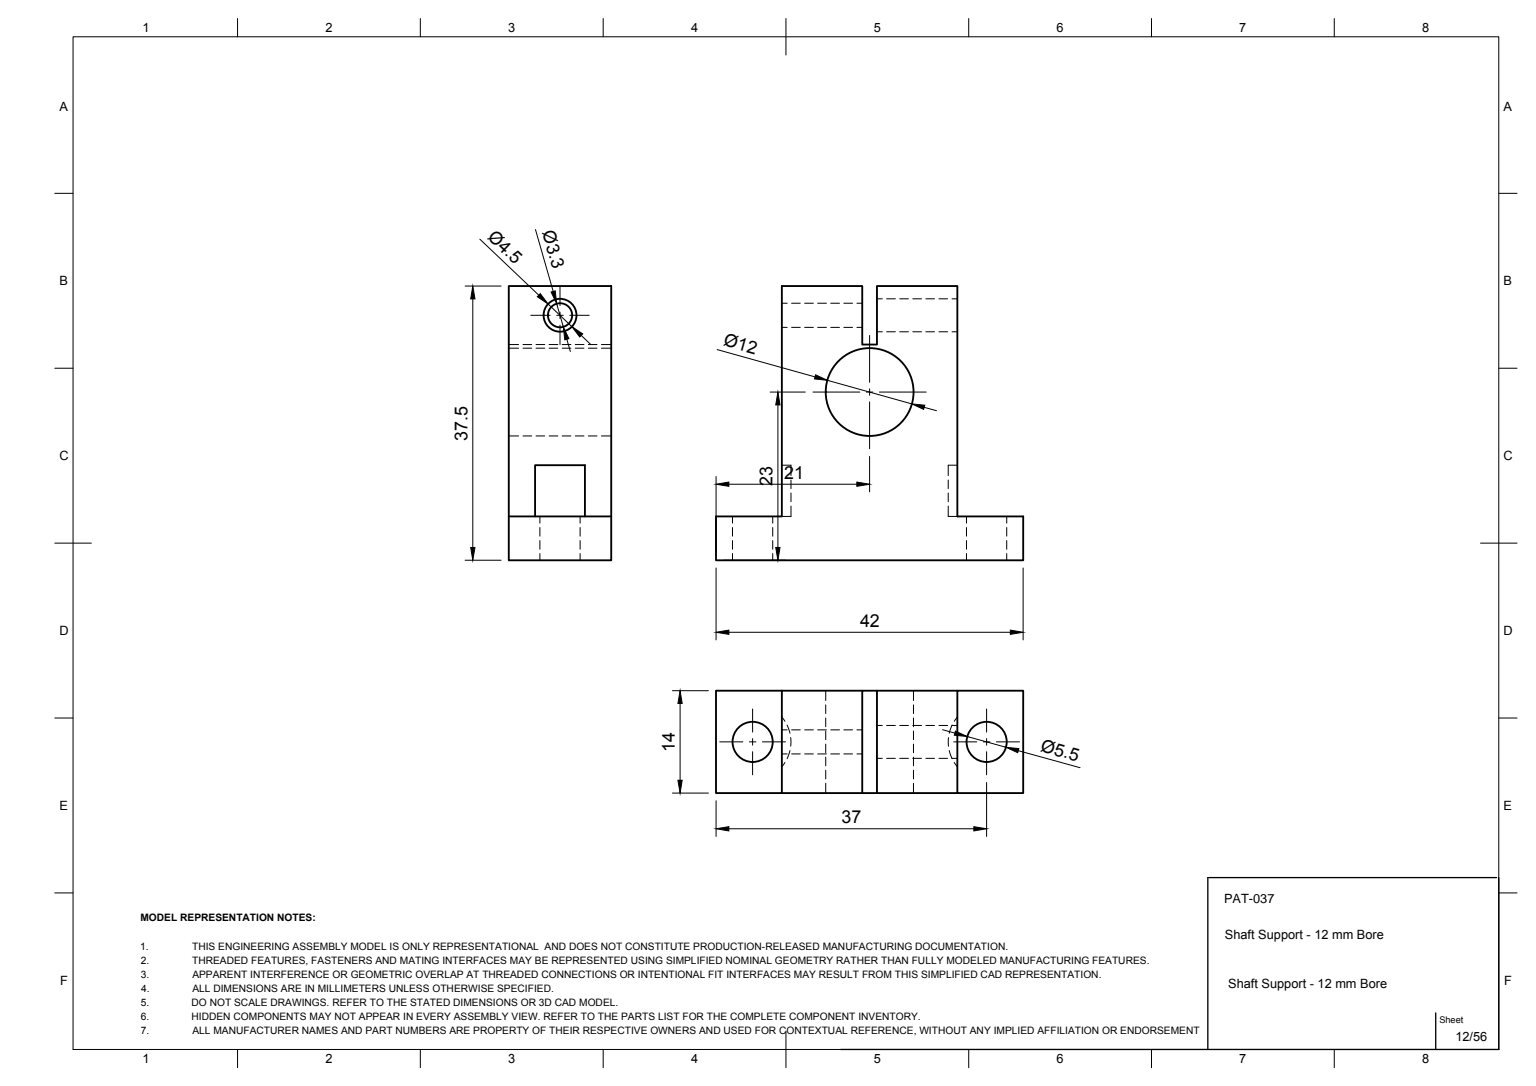
ISO-10303-21;
HEADER;
/* Generated by software containing ST-Developer
 * from STEP Tools, Inc. (www.steptools.com) 
 */

FILE_DESCRIPTION(
/* description */ ('Flywheel Crank-Slider'),
/* implementation_level */ '2;1');

FILE_NAME(
/* name */ 'Shaft Support - 12 mm Bore.step',
/* time_stamp */ '2026-10-28T03:23:13-07:00',
/* author */ (''),
/* organization */ (''),
/* preprocessor_version */ 'ST-DEVELOPER v20.2',
/* originating_system */ 'Autodesk Translation Framework v15.17.0.0',
/* authorisation */ '');

FILE_SCHEMA (('AUTOMOTIVE_DESIGN { 1 0 10303 214 3 1 1 }'));
ENDSEC;

DATA;
#10=MECHANICAL_DESIGN_GEOMETRIC_PRESENTATION_REPRESENTATION('',(#685),#17322);
#580=SHAPE_REPRESENTATION_RELATIONSHIP('SRR','None',#17577,#632);
#632=ADVANCED_BREP_SHAPE_REPRESENTATION('',(#744),#17281);
#685=STYLED_ITEM('',(#17931),#744);
#744=MANIFOLD_SOLID_BREP('Body1',#9065);
#894=FACE_BOUND('',#2179,.T.);
#895=FACE_BOUND('',#2181,.T.);
#896=FACE_BOUND('',#2183,.T.);
#897=FACE_BOUND('',#2190,.T.);
#898=FACE_BOUND('',#2193,.T.);
#899=FACE_BOUND('',#2194,.T.);
#900=FACE_BOUND('',#2197,.T.);
#901=FACE_BOUND('',#2200,.T.);
#902=FACE_BOUND('',#2203,.T.);
#903=FACE_BOUND('',#2206,.T.);
#1133=PLANE('',#10078);
#1134=PLANE('',#10085);
#1135=PLANE('',#10086);
#1136=PLANE('',#10088);
#1137=PLANE('',#10090);
#1138=PLANE('',#10104);
#1139=PLANE('',#10105);
#1140=PLANE('',#10106);
#1141=PLANE('',#10107);
#1142=PLANE('',#10108);
#1143=PLANE('',#10109);
#1144=PLANE('',#10110);
#1145=PLANE('',#10111);
#1146=PLANE('',#10112);
#1147=PLANE('',#10113);
#1148=PLANE('',#10114);
#1530=FACE_OUTER_BOUND('',#2174,.T.);
#1531=FACE_OUTER_BOUND('',#2175,.T.);
#1532=FACE_OUTER_BOUND('',#2176,.T.);
#1533=FACE_OUTER_BOUND('',#2177,.T.);
#1534=FACE_OUTER_BOUND('',#2178,.T.);
#1535=FACE_OUTER_BOUND('',#2180,.T.);
#1536=FACE_OUTER_BOUND('',#2182,.T.);
#1537=FACE_OUTER_BOUND('',#2184,.T.);
#1538=FACE_OUTER_BOUND('',#2185,.T.);
#1539=FACE_OUTER_BOUND('',#2186,.T.);
#1540=FACE_OUTER_BOUND('',#2187,.T.);
#1541=FACE_OUTER_BOUND('',#2188,.T.);
#1542=FACE_OUTER_BOUND('',#2189,.T.);
#1543=FACE_OUTER_BOUND('',#2191,.T.);
#1544=FACE_OUTER_BOUND('',#2192,.T.);
#1545=FACE_OUTER_BOUND('',#2195,.T.);
#1546=FACE_OUTER_BOUND('',#2196,.T.);
#1547=FACE_OUTER_BOUND('',#2198,.T.);
#1548=FACE_OUTER_BOUND('',#2199,.T.);
#1549=FACE_OUTER_BOUND('',#2201,.T.);
#1550=FACE_OUTER_BOUND('',#2202,.T.);
#1551=FACE_OUTER_BOUND('',#2204,.T.);
#1552=FACE_OUTER_BOUND('',#2205,.T.);
#2174=EDGE_LOOP('',(#7002,#7003));
#2175=EDGE_LOOP('',(#7004,#7005,#7006,#7007));
#2176=EDGE_LOOP('',(#7008,#7009,#7010,#7011));
#2177=EDGE_LOOP('',(#7012,#7013));
#2178=EDGE_LOOP('',(#7014,#7015,#7016,#7017,#7018,#7019));
#2179=EDGE_LOOP('',(#7020));
#2180=EDGE_LOOP('',(#7021,#7022,#7023,#7024,#7025,#7026,#7027,#7028));
#2181=EDGE_LOOP('',(#7029));
#2182=EDGE_LOOP('',(#7030,#7031,#7032,#7033,#7034,#7035));
#2183=EDGE_LOOP('',(#7036));
#2184=EDGE_LOOP('',(#7037,#7038,#7039,#7040));
#2185=EDGE_LOOP('',(#7041,#7042,#7043,#7044));
#2186=EDGE_LOOP('',(#7045,#7046,#7047,#7048));
#2187=EDGE_LOOP('',(#7049,#7050,#7051,#7052));
#2188=EDGE_LOOP('',(#7053,#7054,#7055,#7056));
#2189=EDGE_LOOP('',(#7057,#7058,#7059,#7060,#7061,#7062,#7063,#7064,#7065,
#7066,#7067,#7068));
#2190=EDGE_LOOP('',(#7069));
#2191=EDGE_LOOP('',(#7070,#7071,#7072,#7073));
#2192=EDGE_LOOP('',(#7074,#7075,#7076,#7077));
#2193=EDGE_LOOP('',(#7078));
#2194=EDGE_LOOP('',(#7079));
#2195=EDGE_LOOP('',(#7080,#7081,#7082,#7083));
#2196=EDGE_LOOP('',(#7084,#7085,#7086,#7087,#7088,#7089,#7090,#7091));
#2197=EDGE_LOOP('',(#7092));
#2198=EDGE_LOOP('',(#7093,#7094,#7095,#7096));
#2199=EDGE_LOOP('',(#7097,#7098,#7099,#7100));
#2200=EDGE_LOOP('',(#7101));
#2201=EDGE_LOOP('',(#7102,#7103,#7104,#7105));
#2202=EDGE_LOOP('',(#7106,#7107,#7108,#7109));
#2203=EDGE_LOOP('',(#7110));
#2204=EDGE_LOOP('',(#7111,#7112,#7113,#7114));
#2205=EDGE_LOOP('',(#7115,#7116,#7117,#7118,#7119,#7120,#7121,#7122,#7123,
#7124,#7125,#7126));
#2206=EDGE_LOOP('',(#7127));
#2871=LINE('',#15107,#3482);
#2872=LINE('',#15111,#3483);
#2873=LINE('',#15114,#3484);
#2874=LINE('',#15118,#3485);
#2875=LINE('',#15122,#3486);
#2876=LINE('',#15125,#3487);
#2877=LINE('',#15128,#3488);
#2878=LINE('',#15130,#3489);
#2879=LINE('',#15132,#3490);
#2880=LINE('',#15134,#3491);
#2881=LINE('',#15135,#3492);
#2882=LINE('',#15140,#3493);
#2883=LINE('',#15142,#3494);
#2884=LINE('',#15143,#3495);
#2885=LINE('',#15149,#3496);
#2886=LINE('',#15151,#3497);
#2887=LINE('',#15152,#3498);
#2888=LINE('',#15154,#3499);
#2889=LINE('',#15155,#3500);
#2890=LINE('',#15162,#3501);
#2891=LINE('',#15166,#3502);
#2892=LINE('',#15171,#3503);
#2893=LINE('',#15175,#3504);
#2894=LINE('',#15180,#3505);
#2895=LINE('',#15184,#3506);
#2896=LINE('',#15186,#3507);
#2897=LINE('',#15187,#3508);
#2898=LINE('',#15189,#3509);
#2899=LINE('',#15191,#3510);
#2900=LINE('',#15193,#3511);
#2901=LINE('',#15195,#3512);
#2902=LINE('',#15197,#3513);
#2903=LINE('',#15198,#3514);
#2904=LINE('',#15201,#3515);
#2905=LINE('',#15202,#3516);
#2906=LINE('',#15205,#3517);
#2907=LINE('',#15206,#3518);
#2908=LINE('',#15208,#3519);
#2909=LINE('',#15211,#3520);
#2910=LINE('',#15212,#3521);
#2911=LINE('',#15215,#3522);
#2912=LINE('',#15216,#3523);
#2913=LINE('',#15219,#3524);
#2914=LINE('',#15220,#3525);
#2915=LINE('',#15223,#3526);
#2916=LINE('',#15224,#3527);
#2917=LINE('',#15227,#3528);
#2918=LINE('',#15228,#3529);
#2919=LINE('',#15230,#3530);
#3482=VECTOR('',#11873,1.);
#3483=VECTOR('',#11878,1.);
#3484=VECTOR('',#11881,1.);
#3485=VECTOR('',#11884,1.);
#3486=VECTOR('',#11887,1.);
#3487=VECTOR('',#11892,1.);
#3488=VECTOR('',#11895,1.);
#3489=VECTOR('',#11896,1.);
#3490=VECTOR('',#11897,1.);
#3491=VECTOR('',#11898,1.);
#3492=VECTOR('',#11899,1.);
#3493=VECTOR('',#11904,1.);
#3494=VECTOR('',#11905,1.);
#3495=VECTOR('',#11906,1.);
#3496=VECTOR('',#11911,1.);
#3497=VECTOR('',#11912,1.);
#3498=VECTOR('',#11913,1.);
#3499=VECTOR('',#11914,1.);
#3500=VECTOR('',#11915,1.);
#3501=VECTOR('',#11922,0.225);
#3502=VECTOR('',#11927,0.165);
#3503=VECTOR('',#11934,0.275);
#3504=VECTOR('',#11939,0.275);
#3505=VECTOR('',#11944,0.6);
#3506=VECTOR('',#11949,1.);
#3507=VECTOR('',#11950,1.);
#3508=VECTOR('',#11951,1.);
#3509=VECTOR('',#11952,1.);
#3510=VECTOR('',#11953,1.);
#3511=VECTOR('',#11954,1.);
#3512=VECTOR('',#11955,1.);
#3513=VECTOR('',#11956,1.);
#3514=VECTOR('',#11957,1.);
#3515=VECTOR('',#11960,1.);
#3516=VECTOR('',#11961,1.);
#3517=VECTOR('',#11964,1.);
#3518=VECTOR('',#11965,1.);
#3519=VECTOR('',#11968,1.);
#3520=VECTOR('',#11971,1.);
#3521=VECTOR('',#11972,1.);
#3522=VECTOR('',#11975,1.);
#3523=VECTOR('',#11976,1.);
#3524=VECTOR('',#11979,1.);
#3525=VECTOR('',#11980,1.);
#3526=VECTOR('',#11983,1.);
#3527=VECTOR('',#11984,1.);
#3528=VECTOR('',#11987,1.);
#3529=VECTOR('',#11988,1.);
#3530=VECTOR('',#11991,1.);
#3999=CIRCLE('',#10079,0.525);
#4000=CIRCLE('',#10081,0.525);
#4001=CIRCLE('',#10083,0.525);
#4002=CIRCLE('',#10084,0.525);
#4003=CIRCLE('',#10087,0.275);
#4004=CIRCLE('',#10089,0.165);
#4005=CIRCLE('',#10091,0.275);
#4006=CIRCLE('',#10093,0.225);
#4007=CIRCLE('',#10094,0.225);
#4008=CIRCLE('',#10096,0.165);
#4009=CIRCLE('',#10098,0.275);
#4010=CIRCLE('',#10100,0.275);
#4011=CIRCLE('',#10102,0.6);
#4012=CIRCLE('',#10103,0.6);
#4570=VERTEX_POINT('',#15105);
#4571=VERTEX_POINT('',#15106);
#4572=VERTEX_POINT('',#15110);
#4573=VERTEX_POINT('',#15112);
#4574=VERTEX_POINT('',#15116);
#4575=VERTEX_POINT('',#15117);
#4576=VERTEX_POINT('',#15119);
#4577=VERTEX_POINT('',#15121);
#4578=VERTEX_POINT('',#15127);
#4579=VERTEX_POINT('',#15129);
#4580=VERTEX_POINT('',#15131);
#4581=VERTEX_POINT('',#15133);
#4582=VERTEX_POINT('',#15136);
#4583=VERTEX_POINT('',#15139);
#4584=VERTEX_POINT('',#15141);
#4585=VERTEX_POINT('',#15144);
#4586=VERTEX_POINT('',#15147);
#4587=VERTEX_POINT('',#15148);
#4588=VERTEX_POINT('',#15150);
#4589=VERTEX_POINT('',#15153);
#4590=VERTEX_POINT('',#15156);
#4591=VERTEX_POINT('',#15159);
#4592=VERTEX_POINT('',#15161);
#4593=VERTEX_POINT('',#15165);
#4594=VERTEX_POINT('',#15169);
#4595=VERTEX_POINT('',#15173);
#4596=VERTEX_POINT('',#15177);
#4597=VERTEX_POINT('',#15179);
#4598=VERTEX_POINT('',#15183);
#4599=VERTEX_POINT('',#15185);
#4600=VERTEX_POINT('',#15188);
#4601=VERTEX_POINT('',#15190);
#4602=VERTEX_POINT('',#15192);
#4603=VERTEX_POINT('',#15194);
#4604=VERTEX_POINT('',#15196);
#4605=VERTEX_POINT('',#15200);
#4606=VERTEX_POINT('',#15204);
#4607=VERTEX_POINT('',#15210);
#4608=VERTEX_POINT('',#15214);
#4609=VERTEX_POINT('',#15218);
#4610=VERTEX_POINT('',#15222);
#4611=VERTEX_POINT('',#15226);
#5458=EDGE_CURVE('',#4570,#4571,#2871,.T.);
#5459=EDGE_CURVE('',#4571,#4570,#3999,.T.);
#5460=EDGE_CURVE('',#4572,#4570,#2872,.T.);
#5461=EDGE_CURVE('',#4573,#4572,#4000,.T.);
#5462=EDGE_CURVE('',#4571,#4573,#2873,.T.);
#5463=EDGE_CURVE('',#4574,#4575,#2874,.T.);
#5464=EDGE_CURVE('',#4574,#4576,#4001,.T.);
#5465=EDGE_CURVE('',#4577,#4576,#2875,.T.);
#5466=EDGE_CURVE('',#4575,#4577,#4002,.T.);
#5467=EDGE_CURVE('',#4576,#4574,#2876,.T.);
#5468=EDGE_CURVE('',#4572,#4578,#2877,.T.);
#5469=EDGE_CURVE('',#4579,#4578,#2878,.T.);
#5470=EDGE_CURVE('',#4579,#4580,#2879,.T.);
#5471=EDGE_CURVE('',#4581,#4580,#2880,.T.);
#5472=EDGE_CURVE('',#4581,#4573,#2881,.T.);
#5473=EDGE_CURVE('',#4582,#4582,#4003,.T.);
#5474=EDGE_CURVE('',#4583,#4581,#2882,.T.);
#5475=EDGE_CURVE('',#4583,#4584,#2883,.T.);
#5476=EDGE_CURVE('',#4578,#4584,#2884,.T.);
#5477=EDGE_CURVE('',#4585,#4585,#4004,.T.);
#5478=EDGE_CURVE('',#4586,#4587,#2885,.T.);
#5479=EDGE_CURVE('',#4588,#4587,#2886,.T.);
#5480=EDGE_CURVE('',#4575,#4588,#2887,.T.);
#5481=EDGE_CURVE('',#4589,#4577,#2888,.T.);
#5482=EDGE_CURVE('',#4586,#4589,#2889,.T.);
#5483=EDGE_CURVE('',#4590,#4590,#4005,.T.);
#5484=EDGE_CURVE('',#4591,#4591,#4006,.T.);
#5485=EDGE_CURVE('',#4591,#4592,#2890,.T.);
#5486=EDGE_CURVE('',#4592,#4592,#4007,.T.);
#5487=EDGE_CURVE('',#4585,#4593,#2891,.T.);
#5488=EDGE_CURVE('',#4593,#4593,#4008,.T.);
#5489=EDGE_CURVE('',#4594,#4594,#4009,.T.);
#5490=EDGE_CURVE('',#4594,#4582,#2892,.T.);
#5491=EDGE_CURVE('',#4595,#4595,#4010,.T.);
#5492=EDGE_CURVE('',#4595,#4590,#2893,.T.);
#5493=EDGE_CURVE('',#4596,#4596,#4011,.T.);
#5494=EDGE_CURVE('',#4596,#4597,#2894,.T.);
#5495=EDGE_CURVE('',#4597,#4597,#4012,.T.);
#5496=EDGE_CURVE('',#4580,#4598,#2895,.T.);
#5497=EDGE_CURVE('',#4598,#4599,#2896,.T.);
#5498=EDGE_CURVE('',#4599,#4586,#2897,.T.);
#5499=EDGE_CURVE('',#4589,#4600,#2898,.T.);
#5500=EDGE_CURVE('',#4600,#4601,#2899,.T.);
#5501=EDGE_CURVE('',#4601,#4602,#2900,.T.);
#5502=EDGE_CURVE('',#4602,#4603,#2901,.T.);
#5503=EDGE_CURVE('',#4603,#4604,#2902,.T.);
#5504=EDGE_CURVE('',#4604,#4583,#2903,.T.);
#5505=EDGE_CURVE('',#4605,#4579,#2904,.T.);
#5506=EDGE_CURVE('',#4598,#4605,#2905,.T.);
#5507=EDGE_CURVE('',#4606,#4605,#2906,.T.);
#5508=EDGE_CURVE('',#4599,#4606,#2907,.T.);
#5509=EDGE_CURVE('',#4587,#4606,#2908,.T.);
#5510=EDGE_CURVE('',#4607,#4588,#2909,.T.);
#5511=EDGE_CURVE('',#4600,#4607,#2910,.T.);
#5512=EDGE_CURVE('',#4608,#4607,#2911,.T.);
#5513=EDGE_CURVE('',#4601,#4608,#2912,.T.);
#5514=EDGE_CURVE('',#4609,#4608,#2913,.T.);
#5515=EDGE_CURVE('',#4602,#4609,#2914,.T.);
#5516=EDGE_CURVE('',#4610,#4609,#2915,.T.);
#5517=EDGE_CURVE('',#4603,#4610,#2916,.T.);
#5518=EDGE_CURVE('',#4611,#4610,#2917,.T.);
#5519=EDGE_CURVE('',#4604,#4611,#2918,.T.);
#5520=EDGE_CURVE('',#4584,#4611,#2919,.T.);
#7002=ORIENTED_EDGE('',*,*,#5458,.F.);
#7003=ORIENTED_EDGE('',*,*,#5459,.F.);
#7004=ORIENTED_EDGE('',*,*,#5460,.F.);
#7005=ORIENTED_EDGE('',*,*,#5461,.F.);
#7006=ORIENTED_EDGE('',*,*,#5462,.F.);
#7007=ORIENTED_EDGE('',*,*,#5459,.T.);
#7008=ORIENTED_EDGE('',*,*,#5463,.F.);
#7009=ORIENTED_EDGE('',*,*,#5464,.T.);
#7010=ORIENTED_EDGE('',*,*,#5465,.F.);
#7011=ORIENTED_EDGE('',*,*,#5466,.F.);
#7012=ORIENTED_EDGE('',*,*,#5467,.F.);
#7013=ORIENTED_EDGE('',*,*,#5464,.F.);
#7014=ORIENTED_EDGE('',*,*,#5468,.T.);
#7015=ORIENTED_EDGE('',*,*,#5469,.F.);
#7016=ORIENTED_EDGE('',*,*,#5470,.T.);
#7017=ORIENTED_EDGE('',*,*,#5471,.F.);
#7018=ORIENTED_EDGE('',*,*,#5472,.T.);
#7019=ORIENTED_EDGE('',*,*,#5461,.T.);
#7020=ORIENTED_EDGE('',*,*,#5473,.T.);
#7021=ORIENTED_EDGE('',*,*,#5460,.T.);
#7022=ORIENTED_EDGE('',*,*,#5458,.T.);
#7023=ORIENTED_EDGE('',*,*,#5462,.T.);
#7024=ORIENTED_EDGE('',*,*,#5472,.F.);
#7025=ORIENTED_EDGE('',*,*,#5474,.F.);
#7026=ORIENTED_EDGE('',*,*,#5475,.T.);
#7027=ORIENTED_EDGE('',*,*,#5476,.F.);
#7028=ORIENTED_EDGE('',*,*,#5468,.F.);
#7029=ORIENTED_EDGE('',*,*,#5477,.T.);
#7030=ORIENTED_EDGE('',*,*,#5478,.T.);
#7031=ORIENTED_EDGE('',*,*,#5479,.F.);
#7032=ORIENTED_EDGE('',*,*,#5480,.F.);
#7033=ORIENTED_EDGE('',*,*,#5466,.T.);
#7034=ORIENTED_EDGE('',*,*,#5481,.F.);
#7035=ORIENTED_EDGE('',*,*,#5482,.F.);
#7036=ORIENTED_EDGE('',*,*,#5483,.T.);
#7037=ORIENTED_EDGE('',*,*,#5484,.F.);
#7038=ORIENTED_EDGE('',*,*,#5485,.T.);
#7039=ORIENTED_EDGE('',*,*,#5486,.F.);
#7040=ORIENTED_EDGE('',*,*,#5485,.F.);
#7041=ORIENTED_EDGE('',*,*,#5477,.F.);
#7042=ORIENTED_EDGE('',*,*,#5487,.T.);
#7043=ORIENTED_EDGE('',*,*,#5488,.F.);
#7044=ORIENTED_EDGE('',*,*,#5487,.F.);
#7045=ORIENTED_EDGE('',*,*,#5489,.F.);
#7046=ORIENTED_EDGE('',*,*,#5490,.T.);
#7047=ORIENTED_EDGE('',*,*,#5473,.F.);
#7048=ORIENTED_EDGE('',*,*,#5490,.F.);
#7049=ORIENTED_EDGE('',*,*,#5491,.F.);
#7050=ORIENTED_EDGE('',*,*,#5492,.T.);
#7051=ORIENTED_EDGE('',*,*,#5483,.F.);
#7052=ORIENTED_EDGE('',*,*,#5492,.F.);
#7053=ORIENTED_EDGE('',*,*,#5493,.F.);
#7054=ORIENTED_EDGE('',*,*,#5494,.T.);
#7055=ORIENTED_EDGE('',*,*,#5495,.F.);
#7056=ORIENTED_EDGE('',*,*,#5494,.F.);
#7057=ORIENTED_EDGE('',*,*,#5471,.T.);
#7058=ORIENTED_EDGE('',*,*,#5496,.T.);
#7059=ORIENTED_EDGE('',*,*,#5497,.T.);
#7060=ORIENTED_EDGE('',*,*,#5498,.T.);
#7061=ORIENTED_EDGE('',*,*,#5482,.T.);
#7062=ORIENTED_EDGE('',*,*,#5499,.T.);
#7063=ORIENTED_EDGE('',*,*,#5500,.T.);
#7064=ORIENTED_EDGE('',*,*,#5501,.T.);
#7065=ORIENTED_EDGE('',*,*,#5502,.T.);
#7066=ORIENTED_EDGE('',*,*,#5503,.T.);
#7067=ORIENTED_EDGE('',*,*,#5504,.T.);
#7068=ORIENTED_EDGE('',*,*,#5474,.T.);
#7069=ORIENTED_EDGE('',*,*,#5493,.T.);
#7070=ORIENTED_EDGE('',*,*,#5470,.F.);
#7071=ORIENTED_EDGE('',*,*,#5505,.F.);
#7072=ORIENTED_EDGE('',*,*,#5506,.F.);
#7073=ORIENTED_EDGE('',*,*,#5496,.F.);
#7074=ORIENTED_EDGE('',*,*,#5506,.T.);
#7075=ORIENTED_EDGE('',*,*,#5507,.F.);
#7076=ORIENTED_EDGE('',*,*,#5508,.F.);
#7077=ORIENTED_EDGE('',*,*,#5497,.F.);
#7078=ORIENTED_EDGE('',*,*,#5489,.T.);
#7079=ORIENTED_EDGE('',*,*,#5491,.T.);
#7080=ORIENTED_EDGE('',*,*,#5508,.T.);
#7081=ORIENTED_EDGE('',*,*,#5509,.F.);
#7082=ORIENTED_EDGE('',*,*,#5478,.F.);
#7083=ORIENTED_EDGE('',*,*,#5498,.F.);
#7084=ORIENTED_EDGE('',*,*,#5463,.T.);
#7085=ORIENTED_EDGE('',*,*,#5480,.T.);
#7086=ORIENTED_EDGE('',*,*,#5510,.F.);
#7087=ORIENTED_EDGE('',*,*,#5511,.F.);
#7088=ORIENTED_EDGE('',*,*,#5499,.F.);
#7089=ORIENTED_EDGE('',*,*,#5481,.T.);
#7090=ORIENTED_EDGE('',*,*,#5465,.T.);
#7091=ORIENTED_EDGE('',*,*,#5467,.T.);
#7092=ORIENTED_EDGE('',*,*,#5486,.T.);
#7093=ORIENTED_EDGE('',*,*,#5511,.T.);
#7094=ORIENTED_EDGE('',*,*,#5512,.F.);
#7095=ORIENTED_EDGE('',*,*,#5513,.F.);
#7096=ORIENTED_EDGE('',*,*,#5500,.F.);
#7097=ORIENTED_EDGE('',*,*,#5513,.T.);
#7098=ORIENTED_EDGE('',*,*,#5514,.F.);
#7099=ORIENTED_EDGE('',*,*,#5515,.F.);
#7100=ORIENTED_EDGE('',*,*,#5501,.F.);
#7101=ORIENTED_EDGE('',*,*,#5484,.T.);
#7102=ORIENTED_EDGE('',*,*,#5515,.T.);
#7103=ORIENTED_EDGE('',*,*,#5516,.F.);
#7104=ORIENTED_EDGE('',*,*,#5517,.F.);
#7105=ORIENTED_EDGE('',*,*,#5502,.F.);
#7106=ORIENTED_EDGE('',*,*,#5517,.T.);
#7107=ORIENTED_EDGE('',*,*,#5518,.F.);
#7108=ORIENTED_EDGE('',*,*,#5519,.F.);
#7109=ORIENTED_EDGE('',*,*,#5503,.F.);
#7110=ORIENTED_EDGE('',*,*,#5488,.T.);
#7111=ORIENTED_EDGE('',*,*,#5519,.T.);
#7112=ORIENTED_EDGE('',*,*,#5520,.F.);
#7113=ORIENTED_EDGE('',*,*,#5475,.F.);
#7114=ORIENTED_EDGE('',*,*,#5504,.F.);
#7115=ORIENTED_EDGE('',*,*,#5469,.T.);
#7116=ORIENTED_EDGE('',*,*,#5476,.T.);
#7117=ORIENTED_EDGE('',*,*,#5520,.T.);
#7118=ORIENTED_EDGE('',*,*,#5518,.T.);
#7119=ORIENTED_EDGE('',*,*,#5516,.T.);
#7120=ORIENTED_EDGE('',*,*,#5514,.T.);
#7121=ORIENTED_EDGE('',*,*,#5512,.T.);
#7122=ORIENTED_EDGE('',*,*,#5510,.T.);
#7123=ORIENTED_EDGE('',*,*,#5479,.T.);
#7124=ORIENTED_EDGE('',*,*,#5509,.T.);
#7125=ORIENTED_EDGE('',*,*,#5507,.T.);
#7126=ORIENTED_EDGE('',*,*,#5505,.T.);
#7127=ORIENTED_EDGE('',*,*,#5495,.T.);
#8409=CYLINDRICAL_SURFACE('',#10080,0.525);
#8410=CYLINDRICAL_SURFACE('',#10082,0.525);
#8411=CYLINDRICAL_SURFACE('',#10092,0.225);
#8412=CYLINDRICAL_SURFACE('',#10095,0.165);
#8413=CYLINDRICAL_SURFACE('',#10097,0.275);
#8414=CYLINDRICAL_SURFACE('',#10099,0.275);
#8415=CYLINDRICAL_SURFACE('',#10101,0.6);
#8721=ADVANCED_FACE('',(#1530),#1133,.F.);
#8722=ADVANCED_FACE('',(#1531),#8409,.F.);
#8723=ADVANCED_FACE('',(#1532),#8410,.F.);
#8724=ADVANCED_FACE('',(#1533),#1134,.F.);
#8725=ADVANCED_FACE('',(#1534,#894),#1135,.T.);
#8726=ADVANCED_FACE('',(#1535,#895),#1136,.T.);
#8727=ADVANCED_FACE('',(#1536,#896),#1137,.T.);
#8728=ADVANCED_FACE('',(#1537),#8411,.F.);
#8729=ADVANCED_FACE('',(#1538),#8412,.F.);
#8730=ADVANCED_FACE('',(#1539),#8413,.F.);
#8731=ADVANCED_FACE('',(#1540),#8414,.F.);
#8732=ADVANCED_FACE('',(#1541),#8415,.F.);
#8733=ADVANCED_FACE('',(#1542,#897),#1138,.T.);
#8734=ADVANCED_FACE('',(#1543),#1139,.T.);
#8735=ADVANCED_FACE('',(#1544,#898,#899),#1140,.T.);
#8736=ADVANCED_FACE('',(#1545),#1141,.T.);
#8737=ADVANCED_FACE('',(#1546,#900),#1142,.T.);
#8738=ADVANCED_FACE('',(#1547),#1143,.T.);
#8739=ADVANCED_FACE('',(#1548,#901),#1144,.T.);
#8740=ADVANCED_FACE('',(#1549),#1145,.T.);
#8741=ADVANCED_FACE('',(#1550,#902),#1146,.T.);
#8742=ADVANCED_FACE('',(#1551),#1147,.T.);
#8743=ADVANCED_FACE('',(#1552,#903),#1148,.T.);
#9065=CLOSED_SHELL('',(#8721,#8722,#8723,#8724,#8725,#8726,#8727,#8728,
#8729,#8730,#8731,#8732,#8733,#8734,#8735,#8736,#8737,#8738,#8739,#8740,
#8741,#8742,#8743));
#10077=AXIS2_PLACEMENT_3D('',#15103,#11869,#11870);
#10078=AXIS2_PLACEMENT_3D('',#15104,#11871,#11872);
#10079=AXIS2_PLACEMENT_3D('',#15108,#11874,#11875);
#10080=AXIS2_PLACEMENT_3D('',#15109,#11876,#11877);
#10081=AXIS2_PLACEMENT_3D('',#15113,#11879,#11880);
#10082=AXIS2_PLACEMENT_3D('',#15115,#11882,#11883);
#10083=AXIS2_PLACEMENT_3D('',#15120,#11885,#11886);
#10084=AXIS2_PLACEMENT_3D('',#15123,#11888,#11889);
#10085=AXIS2_PLACEMENT_3D('',#15124,#11890,#11891);
#10086=AXIS2_PLACEMENT_3D('',#15126,#11893,#11894);
#10087=AXIS2_PLACEMENT_3D('',#15137,#11900,#11901);
#10088=AXIS2_PLACEMENT_3D('',#15138,#11902,#11903);
#10089=AXIS2_PLACEMENT_3D('',#15145,#11907,#11908);
#10090=AXIS2_PLACEMENT_3D('',#15146,#11909,#11910);
#10091=AXIS2_PLACEMENT_3D('',#15157,#11916,#11917);
#10092=AXIS2_PLACEMENT_3D('',#15158,#11918,#11919);
#10093=AXIS2_PLACEMENT_3D('',#15160,#11920,#11921);
#10094=AXIS2_PLACEMENT_3D('',#15163,#11923,#11924);
#10095=AXIS2_PLACEMENT_3D('',#15164,#11925,#11926);
#10096=AXIS2_PLACEMENT_3D('',#15167,#11928,#11929);
#10097=AXIS2_PLACEMENT_3D('',#15168,#11930,#11931);
#10098=AXIS2_PLACEMENT_3D('',#15170,#11932,#11933);
#10099=AXIS2_PLACEMENT_3D('',#15172,#11935,#11936);
#10100=AXIS2_PLACEMENT_3D('',#15174,#11937,#11938);
#10101=AXIS2_PLACEMENT_3D('',#15176,#11940,#11941);
#10102=AXIS2_PLACEMENT_3D('',#15178,#11942,#11943);
#10103=AXIS2_PLACEMENT_3D('',#15181,#11945,#11946);
#10104=AXIS2_PLACEMENT_3D('',#15182,#11947,#11948);
#10105=AXIS2_PLACEMENT_3D('',#15199,#11958,#11959);
#10106=AXIS2_PLACEMENT_3D('',#15203,#11962,#11963);
#10107=AXIS2_PLACEMENT_3D('',#15207,#11966,#11967);
#10108=AXIS2_PLACEMENT_3D('',#15209,#11969,#11970);
#10109=AXIS2_PLACEMENT_3D('',#15213,#11973,#11974);
#10110=AXIS2_PLACEMENT_3D('',#15217,#11977,#11978);
#10111=AXIS2_PLACEMENT_3D('',#15221,#11981,#11982);
#10112=AXIS2_PLACEMENT_3D('',#15225,#11985,#11986);
#10113=AXIS2_PLACEMENT_3D('',#15229,#11989,#11990);
#10114=AXIS2_PLACEMENT_3D('',#15231,#11992,#11993);
#11869=DIRECTION('axis',(0.,0.,1.));
#11870=DIRECTION('refdir',(1.,0.,0.));
#11871=DIRECTION('center_axis',(0.,0.,1.));
#11872=DIRECTION('ref_axis',(1.,0.,0.));
#11873=DIRECTION('',(0.,-1.,0.));
#11874=DIRECTION('center_axis',(0.,0.,1.));
#11875=DIRECTION('ref_axis',(1.,0.,0.));
#11876=DIRECTION('center_axis',(0.,0.,1.));
#11877=DIRECTION('ref_axis',(1.,0.,0.));
#11878=DIRECTION('',(0.,0.,1.));
#11879=DIRECTION('center_axis',(0.,0.,1.));
#11880=DIRECTION('ref_axis',(1.,0.,0.));
#11881=DIRECTION('',(0.,0.,-1.));
#11882=DIRECTION('center_axis',(0.,0.,1.));
#11883=DIRECTION('ref_axis',(-1.,1.22464679914735E-16,0.));
#11884=DIRECTION('',(0.,0.,-1.));
#11885=DIRECTION('center_axis',(0.,0.,1.));
#11886=DIRECTION('ref_axis',(1.,0.,0.));
#11887=DIRECTION('',(0.,0.,1.));
#11888=DIRECTION('center_axis',(0.,0.,1.));
#11889=DIRECTION('ref_axis',(1.,0.,0.));
#11890=DIRECTION('center_axis',(0.,0.,1.));
#11891=DIRECTION('ref_axis',(1.,0.,0.));
#11892=DIRECTION('',(0.,1.,0.));
#11893=DIRECTION('center_axis',(0.,0.,1.));
#11894=DIRECTION('ref_axis',(1.,0.,0.));
#11895=DIRECTION('',(0.,1.,0.));
#11896=DIRECTION('',(1.,0.,0.));
#11897=DIRECTION('',(0.,-1.,0.));
#11898=DIRECTION('',(-1.,0.,0.));
#11899=DIRECTION('',(0.,1.,0.));
#11900=DIRECTION('center_axis',(0.,0.,-1.));
#11901=DIRECTION('ref_axis',(1.,0.,0.));
#11902=DIRECTION('center_axis',(-1.,0.,0.));
#11903=DIRECTION('ref_axis',(0.,0.,1.));
#11904=DIRECTION('',(0.,0.,-1.));
#11905=DIRECTION('',(0.,1.,0.));
#11906=DIRECTION('',(0.,0.,1.));
#11907=DIRECTION('center_axis',(1.,0.,0.));
#11908=DIRECTION('ref_axis',(0.,0.,-1.));
#11909=DIRECTION('center_axis',(0.,0.,1.));
#11910=DIRECTION('ref_axis',(1.,0.,0.));
#11911=DIRECTION('',(0.,1.,0.));
#11912=DIRECTION('',(1.,0.,0.));
#11913=DIRECTION('',(0.,1.,0.));
#11914=DIRECTION('',(0.,1.,0.));
#11915=DIRECTION('',(-1.,0.,0.));
#11916=DIRECTION('center_axis',(0.,0.,-1.));
#11917=DIRECTION('ref_axis',(1.,0.,0.));
#11918=DIRECTION('center_axis',(1.,0.,0.));
#11919=DIRECTION('ref_axis',(0.,0.,-1.));
#11920=DIRECTION('center_axis',(1.,0.,0.));
#11921=DIRECTION('ref_axis',(0.,0.,-1.));
#11922=DIRECTION('',(1.,0.,0.));
#11923=DIRECTION('center_axis',(-1.,0.,0.));
#11924=DIRECTION('ref_axis',(0.,0.,-1.));
#11925=DIRECTION('center_axis',(1.,0.,0.));
#11926=DIRECTION('ref_axis',(0.,0.,-1.));
#11927=DIRECTION('',(1.,0.,0.));
#11928=DIRECTION('center_axis',(-1.,0.,0.));
#11929=DIRECTION('ref_axis',(0.,0.,-1.));
#11930=DIRECTION('center_axis',(0.,0.,1.));
#11931=DIRECTION('ref_axis',(1.,0.,0.));
#11932=DIRECTION('center_axis',(0.,0.,1.));
#11933=DIRECTION('ref_axis',(1.,0.,0.));
#11934=DIRECTION('',(0.,0.,1.));
#11935=DIRECTION('center_axis',(0.,0.,1.));
#11936=DIRECTION('ref_axis',(1.,0.,0.));
#11937=DIRECTION('center_axis',(0.,0.,1.));
#11938=DIRECTION('ref_axis',(1.,0.,0.));
#11939=DIRECTION('',(0.,0.,1.));
#11940=DIRECTION('center_axis',(0.,1.,0.));
#11941=DIRECTION('ref_axis',(1.,0.,0.));
#11942=DIRECTION('center_axis',(0.,1.,0.));
#11943=DIRECTION('ref_axis',(1.,0.,0.));
#11944=DIRECTION('',(0.,1.,0.));
#11945=DIRECTION('center_axis',(0.,-1.,0.));
#11946=DIRECTION('ref_axis',(1.,0.,0.));
#11947=DIRECTION('center_axis',(0.,-1.,0.));
#11948=DIRECTION('ref_axis',(0.,0.,-1.));
#11949=DIRECTION('',(0.,0.,-1.));
#11950=DIRECTION('',(1.,0.,0.));
#11951=DIRECTION('',(0.,0.,1.));
#11952=DIRECTION('',(0.,0.,1.));
#11953=DIRECTION('',(-1.,0.,0.));
#11954=DIRECTION('',(0.,0.,-1.));
#11955=DIRECTION('',(-1.,0.,0.));
#11956=DIRECTION('',(0.,0.,1.));
#11957=DIRECTION('',(-1.,0.,0.));
#11958=DIRECTION('center_axis',(-1.,0.,0.));
#11959=DIRECTION('ref_axis',(0.,0.,1.));
#11960=DIRECTION('',(0.,0.,1.));
#11961=DIRECTION('',(0.,1.,0.));
#11962=DIRECTION('center_axis',(0.,0.,-1.));
#11963=DIRECTION('ref_axis',(-1.,0.,0.));
#11964=DIRECTION('',(-1.,0.,0.));
#11965=DIRECTION('',(0.,1.,0.));
#11966=DIRECTION('center_axis',(1.,0.,0.));
#11967=DIRECTION('ref_axis',(0.,0.,-1.));
#11968=DIRECTION('',(0.,0.,-1.));
#11969=DIRECTION('center_axis',(1.,0.,0.));
#11970=DIRECTION('ref_axis',(0.,0.,-1.));
#11971=DIRECTION('',(0.,0.,-1.));
#11972=DIRECTION('',(0.,1.,0.));
#11973=DIRECTION('center_axis',(0.,0.,1.));
#11974=DIRECTION('ref_axis',(1.,0.,0.));
#11975=DIRECTION('',(1.,0.,0.));
#11976=DIRECTION('',(0.,1.,0.));
#11977=DIRECTION('center_axis',(-1.,0.,0.));
#11978=DIRECTION('ref_axis',(0.,0.,1.));
#11979=DIRECTION('',(0.,0.,1.));
#11980=DIRECTION('',(0.,1.,0.));
#11981=DIRECTION('center_axis',(0.,0.,1.));
#11982=DIRECTION('ref_axis',(1.,0.,0.));
#11983=DIRECTION('',(1.,0.,0.));
#11984=DIRECTION('',(0.,1.,0.));
#11985=DIRECTION('center_axis',(1.,0.,0.));
#11986=DIRECTION('ref_axis',(0.,0.,-1.));
#11987=DIRECTION('',(0.,0.,-1.));
#11988=DIRECTION('',(0.,1.,0.));
#11989=DIRECTION('center_axis',(0.,0.,1.));
#11990=DIRECTION('ref_axis',(1.,0.,0.));
#11991=DIRECTION('',(1.,0.,0.));
#11992=DIRECTION('center_axis',(0.,1.,0.));
#11993=DIRECTION('ref_axis',(0.,0.,1.));
#15103=CARTESIAN_POINT('',(0.,0.,0.));
#15104=CARTESIAN_POINT('Origin',(-1.6,0.,1.3));
#15105=CARTESIAN_POINT('',(-1.2,0.340036762718386,1.3));
#15106=CARTESIAN_POINT('',(-1.2,-0.340036762718386,1.3));
#15107=CARTESIAN_POINT('',(-1.2,0.,1.3));
#15108=CARTESIAN_POINT('Origin',(-1.6,0.,1.3));
#15109=CARTESIAN_POINT('Origin',(-1.6,0.,0.6));
#15110=CARTESIAN_POINT('',(-1.2,0.340036762718386,0.6));
#15111=CARTESIAN_POINT('',(-1.2,0.340036762718386,0.6));
#15112=CARTESIAN_POINT('',(-1.2,-0.340036762718386,0.6));
#15113=CARTESIAN_POINT('Origin',(-1.6,0.,0.6));
#15114=CARTESIAN_POINT('',(-1.2,-0.340036762718386,0.6));
#15115=CARTESIAN_POINT('Origin',(1.6,0.,0.6));
#15116=CARTESIAN_POINT('',(1.2,0.340036762718386,1.3));
#15117=CARTESIAN_POINT('',(1.2,0.340036762718386,0.6));
#15118=CARTESIAN_POINT('',(1.2,0.340036762718386,0.6));
#15119=CARTESIAN_POINT('',(1.2,-0.340036762718386,1.3));
#15120=CARTESIAN_POINT('Origin',(1.6,0.,1.3));
#15121=CARTESIAN_POINT('',(1.2,-0.340036762718386,0.6));
#15122=CARTESIAN_POINT('',(1.2,-0.340036762718386,0.6));
#15123=CARTESIAN_POINT('Origin',(1.6,0.,0.6));
#15124=CARTESIAN_POINT('Origin',(1.6,0.,1.3));
#15125=CARTESIAN_POINT('',(1.2,0.,1.3));
#15126=CARTESIAN_POINT('Origin',(-2.1,0.,0.6));
#15127=CARTESIAN_POINT('',(-1.2,0.7,0.6));
#15128=CARTESIAN_POINT('',(-1.2,0.,0.6));
#15129=CARTESIAN_POINT('',(-2.1,0.7,0.6));
#15130=CARTESIAN_POINT('',(-1.2,0.7,0.6));
#15131=CARTESIAN_POINT('',(-2.1,-0.7,0.6));
#15132=CARTESIAN_POINT('',(-2.1,0.,0.6));
#15133=CARTESIAN_POINT('',(-1.2,-0.7,0.6));
#15134=CARTESIAN_POINT('',(-1.2,-0.7,0.6));
#15135=CARTESIAN_POINT('',(-1.2,0.,0.6));
#15136=CARTESIAN_POINT('',(-1.875,3.36777869765522E-17,0.6));
#15137=CARTESIAN_POINT('Origin',(-1.6,0.,0.6));
#15138=CARTESIAN_POINT('Origin',(-1.2,0.,0.6));
#15139=CARTESIAN_POINT('',(-1.2,-0.7,3.75));
#15140=CARTESIAN_POINT('',(-1.2,-0.7,3.75));
#15141=CARTESIAN_POINT('',(-1.2,0.7,3.75));
#15142=CARTESIAN_POINT('',(-1.2,0.,3.75));
#15143=CARTESIAN_POINT('',(-1.2,0.7,3.75));
#15144=CARTESIAN_POINT('',(-1.2,-2.02066721859313E-17,3.515));
#15145=CARTESIAN_POINT('Origin',(-1.2,0.,3.35));
#15146=CARTESIAN_POINT('Origin',(1.2,0.,0.6));
#15147=CARTESIAN_POINT('',(2.1,-0.7,0.6));
#15148=CARTESIAN_POINT('',(2.1,0.7,0.6));
#15149=CARTESIAN_POINT('',(2.1,0.,0.6));
#15150=CARTESIAN_POINT('',(1.2,0.7,0.6));
#15151=CARTESIAN_POINT('',(2.1,0.7,0.6));
#15152=CARTESIAN_POINT('',(1.2,0.,0.6));
#15153=CARTESIAN_POINT('',(1.2,-0.7,0.6));
#15154=CARTESIAN_POINT('',(1.2,0.,0.6));
#15155=CARTESIAN_POINT('',(2.1,-0.7,0.6));
#15156=CARTESIAN_POINT('',(1.325,3.36777869765522E-17,0.6));
#15157=CARTESIAN_POINT('Origin',(1.6,0.,0.6));
#15158=CARTESIAN_POINT('Origin',(0.1,0.,3.35));
#15159=CARTESIAN_POINT('',(0.1,-2.75545529808155E-17,3.575));
#15160=CARTESIAN_POINT('Origin',(0.1,0.,3.35));
#15161=CARTESIAN_POINT('',(1.2,2.75545529808155E-17,3.575));
#15162=CARTESIAN_POINT('',(0.1,-2.75545529808155E-17,3.575));
#15163=CARTESIAN_POINT('Origin',(1.2,0.,3.35));
#15164=CARTESIAN_POINT('Origin',(0.,0.,3.35));
#15165=CARTESIAN_POINT('',(-0.1,2.02066721859313E-17,3.515));
#15166=CARTESIAN_POINT('',(0.,-2.02066721859313E-17,3.515));
#15167=CARTESIAN_POINT('Origin',(-0.1,0.,3.35));
#15168=CARTESIAN_POINT('Origin',(-1.6,0.,-0.05));
#15169=CARTESIAN_POINT('',(-1.875,-3.36777869765522E-17,0.));
#15170=CARTESIAN_POINT('Origin',(-1.6,0.,0.));
#15171=CARTESIAN_POINT('',(-1.875,-3.36777869765522E-17,-0.05));
#15172=CARTESIAN_POINT('Origin',(1.6,0.,-0.05));
#15173=CARTESIAN_POINT('',(1.325,-3.36777869765522E-17,0.));
#15174=CARTESIAN_POINT('Origin',(1.6,0.,0.));
#15175=CARTESIAN_POINT('',(1.325,-3.36777869765522E-17,-0.05));
#15176=CARTESIAN_POINT('Origin',(0.,0.,2.3));
#15177=CARTESIAN_POINT('',(-0.6,-0.7,2.3));
#15178=CARTESIAN_POINT('Origin',(0.,-0.7,2.3));
#15179=CARTESIAN_POINT('',(-0.6,0.7,2.3));
#15180=CARTESIAN_POINT('',(-0.6,0.,2.3));
#15181=CARTESIAN_POINT('Origin',(0.,0.7,2.3));
#15182=CARTESIAN_POINT('Origin',(0.,-0.7,1.875));
#15183=CARTESIAN_POINT('',(-2.1,-0.7,0.));
#15184=CARTESIAN_POINT('',(-2.1,-0.7,0.6));
#15185=CARTESIAN_POINT('',(2.1,-0.7,0.));
#15186=CARTESIAN_POINT('',(-2.1,-0.7,0.));
#15187=CARTESIAN_POINT('',(2.1,-0.7,0.));
#15188=CARTESIAN_POINT('',(1.2,-0.7,3.75));
#15189=CARTESIAN_POINT('',(1.2,-0.7,0.6));
#15190=CARTESIAN_POINT('',(0.1,-0.7,3.75));
#15191=CARTESIAN_POINT('',(1.2,-0.7,3.75));
#15192=CARTESIAN_POINT('',(0.1,-0.7,2.95));
#15193=CARTESIAN_POINT('',(0.1,-0.7,3.75));
#15194=CARTESIAN_POINT('',(-0.1,-0.7,2.95));
#15195=CARTESIAN_POINT('',(0.1,-0.7,2.95));
#15196=CARTESIAN_POINT('',(-0.1,-0.7,3.75));
#15197=CARTESIAN_POINT('',(-0.1,-0.7,2.95));
#15198=CARTESIAN_POINT('',(-0.1,-0.7,3.75));
#15199=CARTESIAN_POINT('Origin',(-2.1,0.,0.));
#15200=CARTESIAN_POINT('',(-2.1,0.7,0.));
#15201=CARTESIAN_POINT('',(-2.1,0.7,0.6));
#15202=CARTESIAN_POINT('',(-2.1,0.,0.));
#15203=CARTESIAN_POINT('Origin',(2.1,0.,0.));
#15204=CARTESIAN_POINT('',(2.1,0.7,0.));
#15205=CARTESIAN_POINT('',(-2.1,0.7,0.));
#15206=CARTESIAN_POINT('',(2.1,0.,0.));
#15207=CARTESIAN_POINT('Origin',(2.1,0.,0.6));
#15208=CARTESIAN_POINT('',(2.1,0.7,0.));
#15209=CARTESIAN_POINT('Origin',(1.2,0.,3.75));
#15210=CARTESIAN_POINT('',(1.2,0.7,3.75));
#15211=CARTESIAN_POINT('',(1.2,0.7,0.6));
#15212=CARTESIAN_POINT('',(1.2,0.,3.75));
#15213=CARTESIAN_POINT('Origin',(0.1,0.,3.75));
#15214=CARTESIAN_POINT('',(0.1,0.7,3.75));
#15215=CARTESIAN_POINT('',(1.2,0.7,3.75));
#15216=CARTESIAN_POINT('',(0.1,0.,3.75));
#15217=CARTESIAN_POINT('Origin',(0.1,0.,2.95));
#15218=CARTESIAN_POINT('',(0.1,0.7,2.95));
#15219=CARTESIAN_POINT('',(0.1,0.7,3.75));
#15220=CARTESIAN_POINT('',(0.1,0.,2.95));
#15221=CARTESIAN_POINT('Origin',(-0.1,0.,2.95));
#15222=CARTESIAN_POINT('',(-0.1,0.7,2.95));
#15223=CARTESIAN_POINT('',(0.1,0.7,2.95));
#15224=CARTESIAN_POINT('',(-0.1,0.,2.95));
#15225=CARTESIAN_POINT('Origin',(-0.1,0.,3.75));
#15226=CARTESIAN_POINT('',(-0.1,0.7,3.75));
#15227=CARTESIAN_POINT('',(-0.1,0.7,2.95));
#15228=CARTESIAN_POINT('',(-0.1,0.,3.75));
#15229=CARTESIAN_POINT('Origin',(-1.2,0.,3.75));
#15230=CARTESIAN_POINT('',(-0.1,0.7,3.75));
#15231=CARTESIAN_POINT('Origin',(0.,0.7,1.875));
#17220=UNCERTAINTY_MEASURE_WITH_UNIT(LENGTH_MEASURE(0.001),#17323,
'DISTANCE_ACCURACY_VALUE',
'Maximum model space distance between geometric entities at asserted c
onnectivities');
#17261=UNCERTAINTY_MEASURE_WITH_UNIT(LENGTH_MEASURE(0.001),#17323,
'DISTANCE_ACCURACY_VALUE',
'Maximum model space distance between geometric entities at asserted c
onnectivities');
#17281=(
GEOMETRIC_REPRESENTATION_CONTEXT(3)
GLOBAL_UNCERTAINTY_ASSIGNED_CONTEXT((#17220))
GLOBAL_UNIT_ASSIGNED_CONTEXT((#17323,#17325,#17326))
REPRESENTATION_CONTEXT('','3D')
);
#17322=(
GEOMETRIC_REPRESENTATION_CONTEXT(3)
GLOBAL_UNCERTAINTY_ASSIGNED_CONTEXT((#17261))
GLOBAL_UNIT_ASSIGNED_CONTEXT((#17323,#17325,#17326))
REPRESENTATION_CONTEXT('','3D')
);
#17323=(
LENGTH_UNIT()
NAMED_UNIT(*)
SI_UNIT(.CENTI.,.METRE.)
);
#17325=(
NAMED_UNIT(*)
PLANE_ANGLE_UNIT()
SI_UNIT($,.RADIAN.)
);
#17326=(
NAMED_UNIT(*)
SI_UNIT($,.STERADIAN.)
SOLID_ANGLE_UNIT()
);
#17346=SHAPE_DEFINITION_REPRESENTATION(#17408,#17577);
#17408=PRODUCT_DEFINITION_SHAPE('',$,#17638);
#17577=SHAPE_REPRESENTATION('',(#10077),#17281);
#17618=PRODUCT_DEFINITION_CONTEXT('part definition',#17800,'design');
#17638=PRODUCT_DEFINITION('Shaft Support - 12 mm Bore',
'Shaft Support - 12 mm Bore',#17698,#17618);
#17698=PRODUCT_DEFINITION_FORMATION('',$,#17821);
#17800=APPLICATION_CONTEXT(
'Core Data for Automotive Mechanical Design Process');
#17801=PRODUCT_CONTEXT('part definition',#17800,'mechanical');
#17821=PRODUCT('Shaft Support - 12 mm Bore',
'Shaft Support - 12 mm Bore','Shaft Support - 12 mm Bore',(#17801));
#17925=COLOUR_RGB('Grey',0.48,0.52,0.57);
#17926=FILL_AREA_STYLE_COLOUR('',#17925);
#17927=FILL_AREA_STYLE('',(#17926));
#17928=SURFACE_STYLE_FILL_AREA(#17927);
#17929=SURFACE_SIDE_STYLE('',(#17928));
#17930=SURFACE_STYLE_USAGE(.BOTH.,#17929);
#17931=PRESENTATION_STYLE_ASSIGNMENT((#17930));
ENDSEC;
END-ISO-10303-21;
